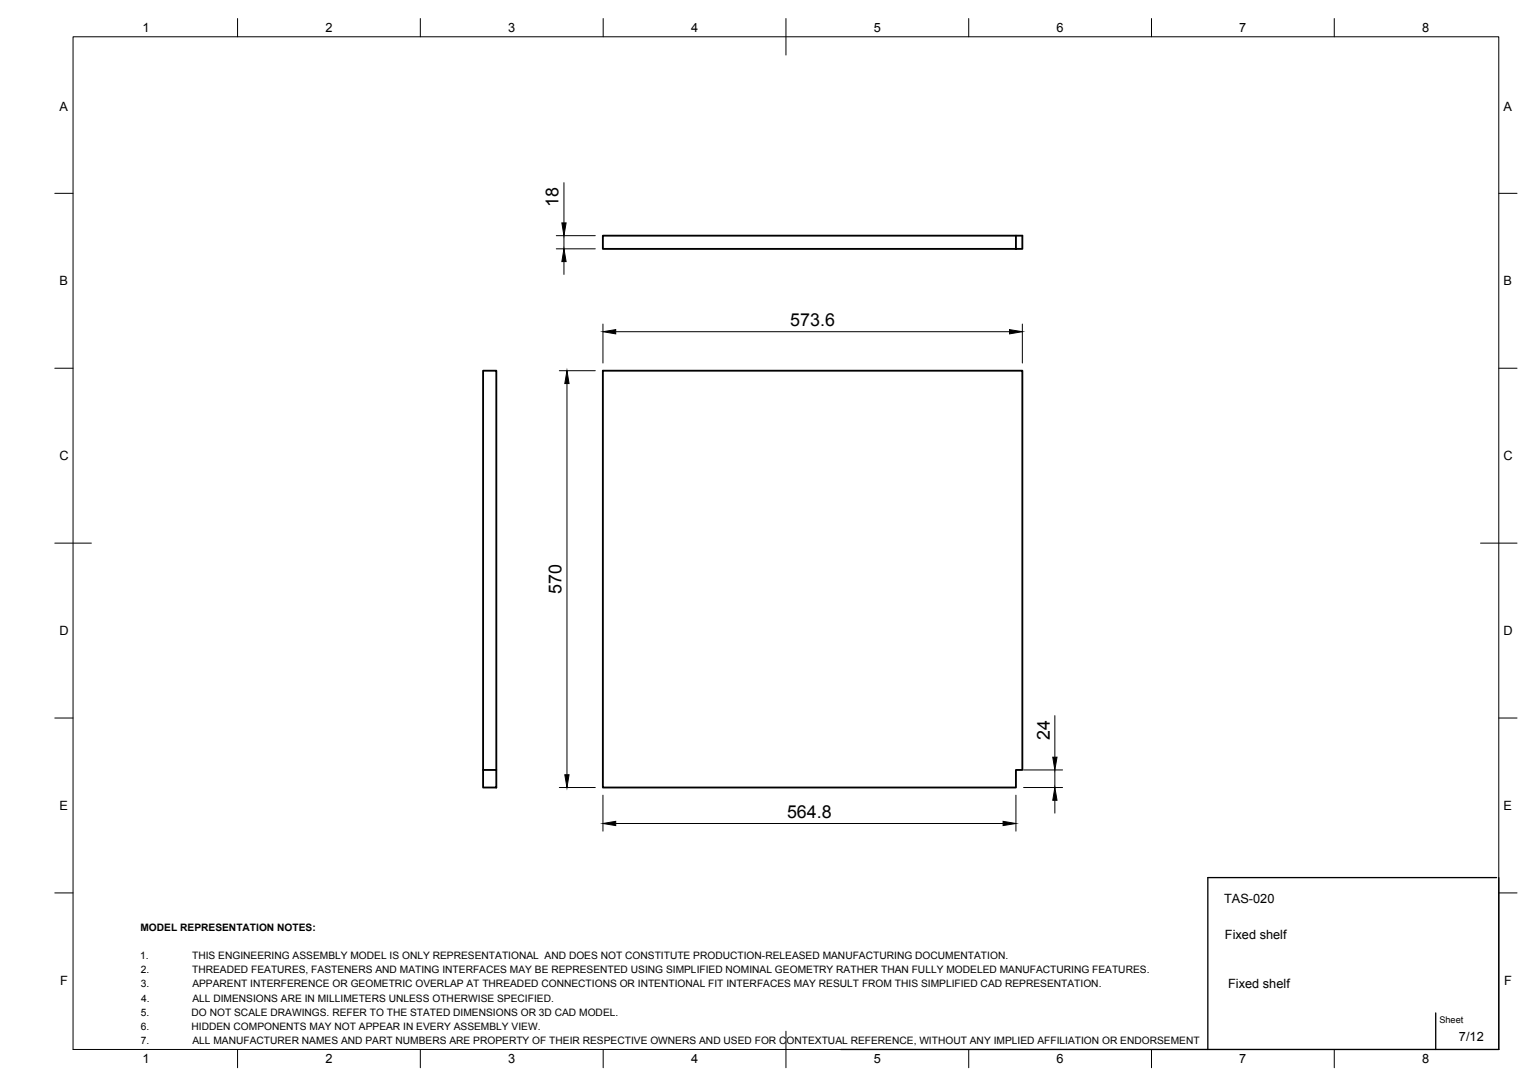
ISO-10303-21;
HEADER;
/* Generated by software containing ST-Developer
 * from STEP Tools, Inc. (www.steptools.com) 
 */

FILE_DESCRIPTION(
/* description */ (''),
/* implementation_level */ '2;1');

FILE_NAME(
/* name */ 'Fixed shelf.step',
/* time_stamp */ '2026-11-15T17:46:57-08:00',
/* author */ (''),
/* organization */ (''),
/* preprocessor_version */ 'ST-DEVELOPER v20.2',
/* originating_system */ 'Autodesk Translation Framework v15.17.0.0',
/* authorisation */ '');

FILE_SCHEMA (('AUTOMOTIVE_DESIGN { 1 0 10303 214 3 1 1 }'));
ENDSEC;

DATA;
#10=MECHANICAL_DESIGN_GEOMETRIC_PRESENTATION_REPRESENTATION('',(#379),#12963);
#355=SHAPE_REPRESENTATION_RELATIONSHIP('SRR','None',#13039,#367);
#367=ADVANCED_BREP_SHAPE_REPRESENTATION('',(#391),#12955);
#379=STYLED_ITEM('',(#13108),#391);
#391=MANIFOLD_SOLID_BREP('Body1',#4813);
#511=PLANE('',#5072);
#512=PLANE('',#5073);
#513=PLANE('',#5074);
#514=PLANE('',#5075);
#515=PLANE('',#5076);
#516=PLANE('',#5077);
#517=PLANE('',#5078);
#518=PLANE('',#5079);
#656=FACE_OUTER_BOUND('',#930,.T.);
#657=FACE_OUTER_BOUND('',#931,.T.);
#658=FACE_OUTER_BOUND('',#932,.T.);
#659=FACE_OUTER_BOUND('',#933,.T.);
#660=FACE_OUTER_BOUND('',#934,.T.);
#661=FACE_OUTER_BOUND('',#935,.T.);
#662=FACE_OUTER_BOUND('',#936,.T.);
#663=FACE_OUTER_BOUND('',#937,.T.);
#930=EDGE_LOOP('',(#3508,#3509,#3510,#3511));
#931=EDGE_LOOP('',(#3512,#3513,#3514,#3515));
#932=EDGE_LOOP('',(#3516,#3517,#3518,#3519));
#933=EDGE_LOOP('',(#3520,#3521,#3522,#3523));
#934=EDGE_LOOP('',(#3524,#3525,#3526,#3527));
#935=EDGE_LOOP('',(#3528,#3529,#3530,#3531));
#936=EDGE_LOOP('',(#3532,#3533,#3534,#3535,#3536,#3537));
#937=EDGE_LOOP('',(#3538,#3539,#3540,#3541,#3542,#3543));
#1296=LINE('',#6940,#1698);
#1297=LINE('',#6942,#1699);
#1298=LINE('',#6944,#1700);
#1299=LINE('',#6945,#1701);
#1300=LINE('',#6948,#1702);
#1301=LINE('',#6950,#1703);
#1302=LINE('',#6951,#1704);
#1303=LINE('',#6954,#1705);
#1304=LINE('',#6956,#1706);
#1305=LINE('',#6957,#1707);
#1306=LINE('',#6960,#1708);
#1307=LINE('',#6962,#1709);
#1308=LINE('',#6963,#1710);
#1309=LINE('',#6966,#1711);
#1310=LINE('',#6968,#1712);
#1311=LINE('',#6969,#1713);
#1312=LINE('',#6971,#1714);
#1313=LINE('',#6972,#1715);
#1698=VECTOR('',#5749,1.);
#1699=VECTOR('',#5750,1.);
#1700=VECTOR('',#5751,1.);
#1701=VECTOR('',#5752,1.);
#1702=VECTOR('',#5755,1.);
#1703=VECTOR('',#5756,1.);
#1704=VECTOR('',#5757,1.);
#1705=VECTOR('',#5760,1.);
#1706=VECTOR('',#5761,1.);
#1707=VECTOR('',#5762,1.);
#1708=VECTOR('',#5765,1.);
#1709=VECTOR('',#5766,1.);
#1710=VECTOR('',#5767,1.);
#1711=VECTOR('',#5770,1.);
#1712=VECTOR('',#5771,1.);
#1713=VECTOR('',#5772,1.);
#1714=VECTOR('',#5775,1.);
#1715=VECTOR('',#5776,1.);
#2144=VERTEX_POINT('',#6938);
#2145=VERTEX_POINT('',#6939);
#2146=VERTEX_POINT('',#6941);
#2147=VERTEX_POINT('',#6943);
#2148=VERTEX_POINT('',#6947);
#2149=VERTEX_POINT('',#6949);
#2150=VERTEX_POINT('',#6953);
#2151=VERTEX_POINT('',#6955);
#2152=VERTEX_POINT('',#6959);
#2153=VERTEX_POINT('',#6961);
#2154=VERTEX_POINT('',#6965);
#2155=VERTEX_POINT('',#6967);
#2650=EDGE_CURVE('',#2144,#2145,#1296,.T.);
#2651=EDGE_CURVE('',#2144,#2146,#1297,.T.);
#2652=EDGE_CURVE('',#2147,#2146,#1298,.T.);
#2653=EDGE_CURVE('',#2145,#2147,#1299,.T.);
#2654=EDGE_CURVE('',#2148,#2144,#1300,.T.);
#2655=EDGE_CURVE('',#2149,#2148,#1301,.T.);
#2656=EDGE_CURVE('',#2146,#2149,#1302,.T.);
#2657=EDGE_CURVE('',#2150,#2147,#1303,.T.);
#2658=EDGE_CURVE('',#2151,#2150,#1304,.T.);
#2659=EDGE_CURVE('',#2151,#2145,#1305,.T.);
#2660=EDGE_CURVE('',#2148,#2152,#1306,.T.);
#2661=EDGE_CURVE('',#2152,#2153,#1307,.T.);
#2662=EDGE_CURVE('',#2149,#2153,#1308,.T.);
#2663=EDGE_CURVE('',#2154,#2151,#1309,.T.);
#2664=EDGE_CURVE('',#2155,#2150,#1310,.T.);
#2665=EDGE_CURVE('',#2154,#2155,#1311,.T.);
#2666=EDGE_CURVE('',#2152,#2154,#1312,.T.);
#2667=EDGE_CURVE('',#2153,#2155,#1313,.T.);
#3508=ORIENTED_EDGE('',*,*,#2650,.F.);
#3509=ORIENTED_EDGE('',*,*,#2651,.T.);
#3510=ORIENTED_EDGE('',*,*,#2652,.F.);
#3511=ORIENTED_EDGE('',*,*,#2653,.F.);
#3512=ORIENTED_EDGE('',*,*,#2654,.F.);
#3513=ORIENTED_EDGE('',*,*,#2655,.F.);
#3514=ORIENTED_EDGE('',*,*,#2656,.F.);
#3515=ORIENTED_EDGE('',*,*,#2651,.F.);
#3516=ORIENTED_EDGE('',*,*,#2653,.T.);
#3517=ORIENTED_EDGE('',*,*,#2657,.F.);
#3518=ORIENTED_EDGE('',*,*,#2658,.F.);
#3519=ORIENTED_EDGE('',*,*,#2659,.T.);
#3520=ORIENTED_EDGE('',*,*,#2655,.T.);
#3521=ORIENTED_EDGE('',*,*,#2660,.T.);
#3522=ORIENTED_EDGE('',*,*,#2661,.T.);
#3523=ORIENTED_EDGE('',*,*,#2662,.F.);
#3524=ORIENTED_EDGE('',*,*,#2663,.T.);
#3525=ORIENTED_EDGE('',*,*,#2658,.T.);
#3526=ORIENTED_EDGE('',*,*,#2664,.F.);
#3527=ORIENTED_EDGE('',*,*,#2665,.F.);
#3528=ORIENTED_EDGE('',*,*,#2666,.T.);
#3529=ORIENTED_EDGE('',*,*,#2665,.T.);
#3530=ORIENTED_EDGE('',*,*,#2667,.F.);
#3531=ORIENTED_EDGE('',*,*,#2661,.F.);
#3532=ORIENTED_EDGE('',*,*,#2656,.T.);
#3533=ORIENTED_EDGE('',*,*,#2662,.T.);
#3534=ORIENTED_EDGE('',*,*,#2667,.T.);
#3535=ORIENTED_EDGE('',*,*,#2664,.T.);
#3536=ORIENTED_EDGE('',*,*,#2657,.T.);
#3537=ORIENTED_EDGE('',*,*,#2652,.T.);
#3538=ORIENTED_EDGE('',*,*,#2650,.T.);
#3539=ORIENTED_EDGE('',*,*,#2659,.F.);
#3540=ORIENTED_EDGE('',*,*,#2663,.F.);
#3541=ORIENTED_EDGE('',*,*,#2666,.F.);
#3542=ORIENTED_EDGE('',*,*,#2660,.F.);
#3543=ORIENTED_EDGE('',*,*,#2654,.T.);
#4637=ADVANCED_FACE('',(#656),#511,.F.);
#4638=ADVANCED_FACE('',(#657),#512,.F.);
#4639=ADVANCED_FACE('',(#658),#513,.T.);
#4640=ADVANCED_FACE('',(#659),#514,.T.);
#4641=ADVANCED_FACE('',(#660),#515,.T.);
#4642=ADVANCED_FACE('',(#661),#516,.T.);
#4643=ADVANCED_FACE('',(#662),#517,.T.);
#4644=ADVANCED_FACE('',(#663),#518,.F.);
#4813=CLOSED_SHELL('',(#4637,#4638,#4639,#4640,#4641,#4642,#4643,#4644));
#5071=AXIS2_PLACEMENT_3D('',#6936,#5745,#5746);
#5072=AXIS2_PLACEMENT_3D('',#6937,#5747,#5748);
#5073=AXIS2_PLACEMENT_3D('',#6946,#5753,#5754);
#5074=AXIS2_PLACEMENT_3D('',#6952,#5758,#5759);
#5075=AXIS2_PLACEMENT_3D('',#6958,#5763,#5764);
#5076=AXIS2_PLACEMENT_3D('',#6964,#5768,#5769);
#5077=AXIS2_PLACEMENT_3D('',#6970,#5773,#5774);
#5078=AXIS2_PLACEMENT_3D('',#6973,#5777,#5778);
#5079=AXIS2_PLACEMENT_3D('',#6974,#5779,#5780);
#5745=DIRECTION('axis',(0.,0.,1.));
#5746=DIRECTION('refdir',(1.,0.,0.));
#5747=DIRECTION('center_axis',(0.,1.,0.));
#5748=DIRECTION('ref_axis',(-1.,0.,0.));
#5749=DIRECTION('',(-1.,0.,0.));
#5750=DIRECTION('',(0.,0.,1.));
#5751=DIRECTION('',(1.,0.,0.));
#5752=DIRECTION('',(0.,0.,1.));
#5753=DIRECTION('center_axis',(1.,0.,0.));
#5754=DIRECTION('ref_axis',(0.,1.,0.));
#5755=DIRECTION('',(0.,1.,0.));
#5756=DIRECTION('',(0.,0.,-1.));
#5757=DIRECTION('',(0.,-1.,0.));
#5758=DIRECTION('center_axis',(-1.,0.,0.));
#5759=DIRECTION('ref_axis',(0.,-1.,0.));
#5760=DIRECTION('',(0.,-1.,0.));
#5761=DIRECTION('',(0.,0.,1.));
#5762=DIRECTION('',(0.,-1.,0.));
#5763=DIRECTION('center_axis',(0.,-1.,0.));
#5764=DIRECTION('ref_axis',(1.,0.,0.));
#5765=DIRECTION('',(1.,0.,0.));
#5766=DIRECTION('',(0.,0.,1.));
#5767=DIRECTION('',(1.,0.,0.));
#5768=DIRECTION('center_axis',(0.,1.,0.));
#5769=DIRECTION('ref_axis',(-1.,0.,0.));
#5770=DIRECTION('',(-1.,0.,0.));
#5771=DIRECTION('',(-1.,0.,0.));
#5772=DIRECTION('',(0.,0.,1.));
#5773=DIRECTION('center_axis',(1.,0.,0.));
#5774=DIRECTION('ref_axis',(0.,1.,0.));
#5775=DIRECTION('',(0.,1.,0.));
#5776=DIRECTION('',(0.,1.,0.));
#5777=DIRECTION('center_axis',(0.,0.,1.));
#5778=DIRECTION('ref_axis',(1.,0.,0.));
#5779=DIRECTION('center_axis',(0.,0.,1.));
#5780=DIRECTION('ref_axis',(1.,0.,0.));
#6936=CARTESIAN_POINT('',(0.,0.,0.));
#6937=CARTESIAN_POINT('Origin',(0.88,3.,0.));
#6938=CARTESIAN_POINT('',(0.88,3.,0.));
#6939=CARTESIAN_POINT('',(0.,3.,0.));
#6940=CARTESIAN_POINT('',(14.78,3.,0.));
#6941=CARTESIAN_POINT('',(0.88,3.,1.8));
#6942=CARTESIAN_POINT('',(0.88,3.,0.));
#6943=CARTESIAN_POINT('',(0.,3.,1.8));
#6944=CARTESIAN_POINT('',(14.78,3.,1.8));
#6945=CARTESIAN_POINT('',(0.,3.,0.));
#6946=CARTESIAN_POINT('Origin',(0.88,0.6,0.));
#6947=CARTESIAN_POINT('',(0.88,0.6,0.));
#6948=CARTESIAN_POINT('',(0.879999999999999,14.85,0.));
#6949=CARTESIAN_POINT('',(0.88,0.6,1.8));
#6950=CARTESIAN_POINT('',(0.88,0.6,0.));
#6951=CARTESIAN_POINT('',(0.879999999999999,14.85,1.8));
#6952=CARTESIAN_POINT('Origin',(0.,57.6,0.));
#6953=CARTESIAN_POINT('',(0.,57.6,1.8));
#6954=CARTESIAN_POINT('',(0.,57.6,1.8));
#6955=CARTESIAN_POINT('',(0.,57.6,0.));
#6956=CARTESIAN_POINT('',(0.,57.6,0.));
#6957=CARTESIAN_POINT('',(0.,57.6,0.));
#6958=CARTESIAN_POINT('Origin',(0.,0.6,0.));
#6959=CARTESIAN_POINT('',(57.36,0.6,0.));
#6960=CARTESIAN_POINT('',(0.,0.6,0.));
#6961=CARTESIAN_POINT('',(57.36,0.600000000000001,1.8));
#6962=CARTESIAN_POINT('',(57.36,0.6,0.));
#6963=CARTESIAN_POINT('',(0.,0.6,1.8));
#6964=CARTESIAN_POINT('Origin',(57.36,57.6,0.));
#6965=CARTESIAN_POINT('',(57.36,57.6,0.));
#6966=CARTESIAN_POINT('',(57.36,57.6,0.));
#6967=CARTESIAN_POINT('',(57.36,57.6,1.8));
#6968=CARTESIAN_POINT('',(57.36,57.6,1.8));
#6969=CARTESIAN_POINT('',(57.36,57.6,0.));
#6970=CARTESIAN_POINT('Origin',(57.36,0.6,0.));
#6971=CARTESIAN_POINT('',(57.36,0.6,0.));
#6972=CARTESIAN_POINT('',(57.36,0.6,1.8));
#6973=CARTESIAN_POINT('Origin',(28.68,29.1,1.8));
#6974=CARTESIAN_POINT('Origin',(28.68,29.1,0.));
#12941=UNCERTAINTY_MEASURE_WITH_UNIT(LENGTH_MEASURE(0.001),#12964,
'DISTANCE_ACCURACY_VALUE',
'Maximum model space distance between geometric entities at asserted c
onnectivities');
#12949=UNCERTAINTY_MEASURE_WITH_UNIT(LENGTH_MEASURE(0.001),#12964,
'DISTANCE_ACCURACY_VALUE',
'Maximum model space distance between geometric entities at asserted c
onnectivities');
#12955=(
GEOMETRIC_REPRESENTATION_CONTEXT(3)
GLOBAL_UNCERTAINTY_ASSIGNED_CONTEXT((#12941))
GLOBAL_UNIT_ASSIGNED_CONTEXT((#12964,#12966,#12967))
REPRESENTATION_CONTEXT('','3D')
);
#12963=(
GEOMETRIC_REPRESENTATION_CONTEXT(3)
GLOBAL_UNCERTAINTY_ASSIGNED_CONTEXT((#12949))
GLOBAL_UNIT_ASSIGNED_CONTEXT((#12964,#12966,#12967))
REPRESENTATION_CONTEXT('','3D')
);
#12964=(
LENGTH_UNIT()
NAMED_UNIT(*)
SI_UNIT(.CENTI.,.METRE.)
);
#12966=(
NAMED_UNIT(*)
PLANE_ANGLE_UNIT()
SI_UNIT($,.RADIAN.)
);
#12967=(
NAMED_UNIT(*)
SI_UNIT($,.STERADIAN.)
SOLID_ANGLE_UNIT()
);
#12973=SHAPE_DEFINITION_REPRESENTATION(#12986,#13039);
#12986=PRODUCT_DEFINITION_SHAPE('',$,#13053);
#13039=SHAPE_REPRESENTATION('',(#5071),#12955);
#13047=PRODUCT_DEFINITION_CONTEXT('part definition',#13088,'design');
#13053=PRODUCT_DEFINITION('Fixed shelf','Fixed shelf',#13066,#13047);
#13066=PRODUCT_DEFINITION_FORMATION('',$,#13095);
#13088=APPLICATION_CONTEXT(
'Core Data for Automotive Mechanical Design Process');
#13089=PRODUCT_CONTEXT('part definition',#13088,'mechanical');
#13095=PRODUCT('Fixed shelf','Fixed shelf',$,(#13089));
#13108=PRESENTATION_STYLE_ASSIGNMENT((#13121));
#13121=SURFACE_STYLE_USAGE(.BOTH.,#13134);
#13134=SURFACE_SIDE_STYLE('',(#13147));
#13147=SURFACE_STYLE_FILL_AREA(#13160);
#13160=FILL_AREA_STYLE('Fixed shelf finish',(#13173));
#13173=FILL_AREA_STYLE_COLOUR('Fixed shelf finish',#13186);
#13186=COLOUR_RGB('Fixed shelf finish',0.274509803921569,0.6,0.8);
ENDSEC;
END-ISO-10303-21;
